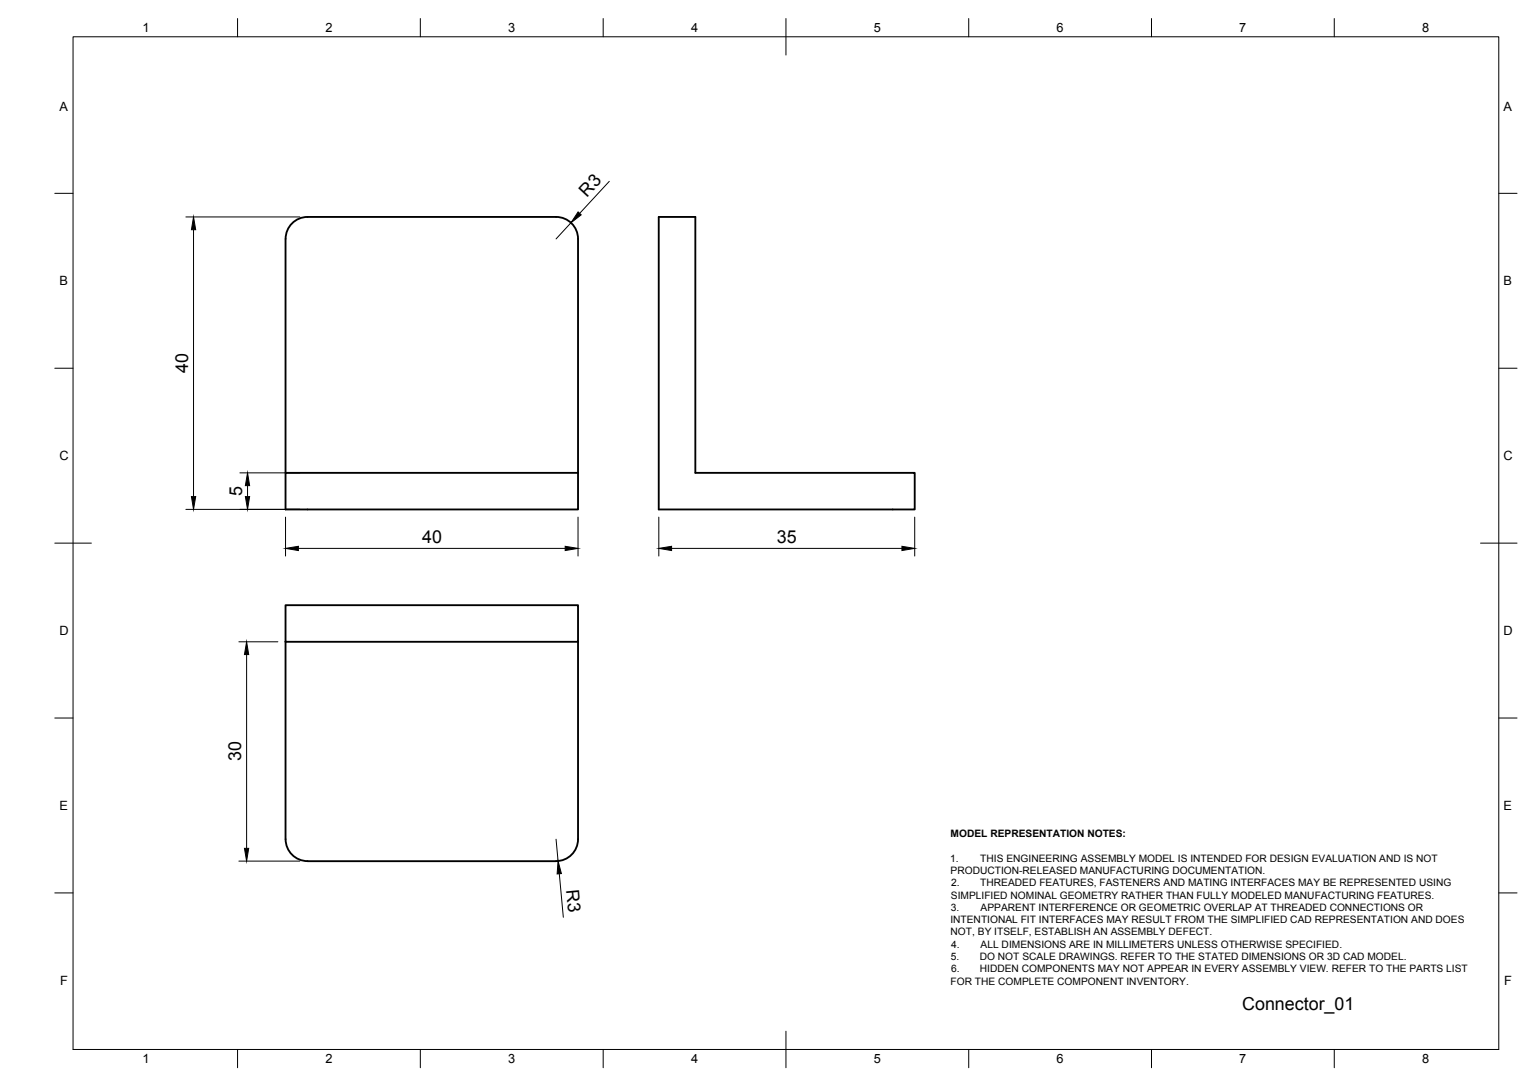
ISO-10303-21;
HEADER;
/* Generated by software containing ST-Developer
 * from STEP Tools, Inc. (www.steptools.com) 
 */

FILE_DESCRIPTION(
/* description */ (''),
/* implementation_level */ '2;1');

FILE_NAME(
/* name */ 'Connector_01.step',
/* time_stamp */ '2026-10-05T19:45:59-07:00',
/* author */ (''),
/* organization */ (''),
/* preprocessor_version */ 'ST-DEVELOPER v20.2',
/* originating_system */ 'Autodesk Translation Framework v15.15.0.0',
/* authorisation */ '');

FILE_SCHEMA (('AUTOMOTIVE_DESIGN { 1 0 10303 214 3 1 1 }'));
ENDSEC;

DATA;
#10=MECHANICAL_DESIGN_GEOMETRIC_PRESENTATION_REPRESENTATION('',(#91),#2462);
#73=SHAPE_REPRESENTATION_RELATIONSHIP('SRR','None',#2499,#82);
#82=ADVANCED_BREP_SHAPE_REPRESENTATION('',(#100),#2454);
#91=STYLED_ITEM('',(#2552),#100);
#100=MANIFOLD_SOLID_BREP('Body1',#1328);
#110=PLANE('',#1447);
#111=PLANE('',#1449);
#112=PLANE('',#1455);
#113=PLANE('',#1456);
#114=PLANE('',#1460);
#115=PLANE('',#1461);
#116=PLANE('',#1462);
#117=PLANE('',#1463);
#168=FACE_OUTER_BOUND('',#248,.T.);
#169=FACE_OUTER_BOUND('',#249,.T.);
#170=FACE_OUTER_BOUND('',#250,.T.);
#171=FACE_OUTER_BOUND('',#251,.T.);
#172=FACE_OUTER_BOUND('',#252,.T.);
#173=FACE_OUTER_BOUND('',#253,.T.);
#174=FACE_OUTER_BOUND('',#254,.T.);
#175=FACE_OUTER_BOUND('',#255,.T.);
#176=FACE_OUTER_BOUND('',#256,.T.);
#177=FACE_OUTER_BOUND('',#257,.T.);
#178=FACE_OUTER_BOUND('',#258,.T.);
#179=FACE_OUTER_BOUND('',#259,.T.);
#248=EDGE_LOOP('',(#900,#901,#902,#903));
#249=EDGE_LOOP('',(#904,#905,#906,#907,#908,#909));
#250=EDGE_LOOP('',(#910,#911,#912,#913));
#251=EDGE_LOOP('',(#914,#915,#916,#917));
#252=EDGE_LOOP('',(#918,#919,#920,#921));
#253=EDGE_LOOP('',(#922,#923,#924,#925));
#254=EDGE_LOOP('',(#926,#927,#928,#929,#930,#931));
#255=EDGE_LOOP('',(#932,#933,#934,#935));
#256=EDGE_LOOP('',(#936,#937,#938,#939,#940,#941));
#257=EDGE_LOOP('',(#942,#943,#944,#945,#946,#947));
#258=EDGE_LOOP('',(#948,#949,#950,#951,#952,#953));
#259=EDGE_LOOP('',(#954,#955,#956,#957,#958,#959));
#341=LINE('',#2000,#460);
#342=LINE('',#2003,#461);
#343=LINE('',#2006,#462);
#344=LINE('',#2010,#463);
#345=LINE('',#2012,#464);
#346=LINE('',#2013,#465);
#347=LINE('',#2016,#466);
#348=LINE('',#2017,#467);
#349=LINE('',#2021,#468);
#350=LINE('',#2027,#469);
#351=LINE('',#2030,#470);
#352=LINE('',#2033,#471);
#353=LINE('',#2035,#472);
#354=LINE('',#2036,#473);
#355=LINE('',#2039,#474);
#356=LINE('',#2041,#475);
#357=LINE('',#2043,#476);
#358=LINE('',#2048,#477);
#359=LINE('',#2050,#478);
#360=LINE('',#2051,#479);
#361=LINE('',#2053,#480);
#362=LINE('',#2055,#481);
#460=VECTOR('',#1600,10.);
#461=VECTOR('',#1603,10.);
#462=VECTOR('',#1606,10.);
#463=VECTOR('',#1609,10.);
#464=VECTOR('',#1610,10.);
#465=VECTOR('',#1611,10.);
#466=VECTOR('',#1614,10.);
#467=VECTOR('',#1615,10.);
#468=VECTOR('',#1620,10.);
#469=VECTOR('',#1625,10.);
#470=VECTOR('',#1628,10.);
#471=VECTOR('',#1631,10.);
#472=VECTOR('',#1632,10.);
#473=VECTOR('',#1633,10.);
#474=VECTOR('',#1636,10.);
#475=VECTOR('',#1637,10.);
#476=VECTOR('',#1638,10.);
#477=VECTOR('',#1645,10.);
#478=VECTOR('',#1648,10.);
#479=VECTOR('',#1649,10.);
#480=VECTOR('',#1652,10.);
#481=VECTOR('',#1655,10.);
#580=CIRCLE('',#1445,3.);
#581=CIRCLE('',#1446,3.);
#582=CIRCLE('',#1448,3.);
#583=CIRCLE('',#1451,3.);
#584=CIRCLE('',#1453,3.);
#585=CIRCLE('',#1454,3.);
#586=CIRCLE('',#1457,3.);
#587=CIRCLE('',#1459,3.);
#623=VERTEX_POINT('',#1996);
#624=VERTEX_POINT('',#1997);
#625=VERTEX_POINT('',#1999);
#626=VERTEX_POINT('',#2001);
#627=VERTEX_POINT('',#2005);
#628=VERTEX_POINT('',#2007);
#629=VERTEX_POINT('',#2009);
#630=VERTEX_POINT('',#2011);
#631=VERTEX_POINT('',#2015);
#632=VERTEX_POINT('',#2019);
#633=VERTEX_POINT('',#2023);
#634=VERTEX_POINT('',#2024);
#635=VERTEX_POINT('',#2026);
#636=VERTEX_POINT('',#2028);
#637=VERTEX_POINT('',#2032);
#638=VERTEX_POINT('',#2034);
#639=VERTEX_POINT('',#2038);
#640=VERTEX_POINT('',#2040);
#641=VERTEX_POINT('',#2042);
#642=VERTEX_POINT('',#2046);
#731=EDGE_CURVE('',#623,#624,#580,.T.);
#732=EDGE_CURVE('',#624,#625,#341,.T.);
#733=EDGE_CURVE('',#625,#626,#581,.T.);
#734=EDGE_CURVE('',#626,#623,#342,.T.);
#735=EDGE_CURVE('',#627,#625,#343,.T.);
#736=EDGE_CURVE('',#628,#627,#582,.T.);
#737=EDGE_CURVE('',#629,#628,#344,.T.);
#738=EDGE_CURVE('',#629,#630,#345,.T.);
#739=EDGE_CURVE('',#630,#626,#346,.T.);
#740=EDGE_CURVE('',#624,#631,#347,.T.);
#741=EDGE_CURVE('',#627,#631,#348,.T.);
#742=EDGE_CURVE('',#631,#632,#583,.T.);
#743=EDGE_CURVE('',#632,#628,#349,.T.);
#744=EDGE_CURVE('',#633,#634,#584,.T.);
#745=EDGE_CURVE('',#634,#635,#350,.T.);
#746=EDGE_CURVE('',#635,#636,#585,.T.);
#747=EDGE_CURVE('',#636,#633,#351,.T.);
#748=EDGE_CURVE('',#637,#636,#352,.T.);
#749=EDGE_CURVE('',#638,#637,#353,.T.);
#750=EDGE_CURVE('',#633,#638,#354,.T.);
#751=EDGE_CURVE('',#639,#635,#355,.T.);
#752=EDGE_CURVE('',#640,#639,#356,.T.);
#753=EDGE_CURVE('',#641,#640,#357,.T.);
#754=EDGE_CURVE('',#637,#641,#586,.T.);
#755=EDGE_CURVE('',#642,#638,#587,.T.);
#756=EDGE_CURVE('',#641,#642,#358,.T.);
#757=EDGE_CURVE('',#642,#630,#359,.T.);
#758=EDGE_CURVE('',#629,#634,#360,.T.);
#759=EDGE_CURVE('',#639,#632,#361,.T.);
#760=EDGE_CURVE('',#640,#623,#362,.T.);
#900=ORIENTED_EDGE('',*,*,#731,.T.);
#901=ORIENTED_EDGE('',*,*,#732,.T.);
#902=ORIENTED_EDGE('',*,*,#733,.T.);
#903=ORIENTED_EDGE('',*,*,#734,.T.);
#904=ORIENTED_EDGE('',*,*,#733,.F.);
#905=ORIENTED_EDGE('',*,*,#735,.F.);
#906=ORIENTED_EDGE('',*,*,#736,.F.);
#907=ORIENTED_EDGE('',*,*,#737,.F.);
#908=ORIENTED_EDGE('',*,*,#738,.T.);
#909=ORIENTED_EDGE('',*,*,#739,.T.);
#910=ORIENTED_EDGE('',*,*,#732,.F.);
#911=ORIENTED_EDGE('',*,*,#740,.T.);
#912=ORIENTED_EDGE('',*,*,#741,.F.);
#913=ORIENTED_EDGE('',*,*,#735,.T.);
#914=ORIENTED_EDGE('',*,*,#736,.T.);
#915=ORIENTED_EDGE('',*,*,#741,.T.);
#916=ORIENTED_EDGE('',*,*,#742,.T.);
#917=ORIENTED_EDGE('',*,*,#743,.T.);
#918=ORIENTED_EDGE('',*,*,#744,.T.);
#919=ORIENTED_EDGE('',*,*,#745,.T.);
#920=ORIENTED_EDGE('',*,*,#746,.T.);
#921=ORIENTED_EDGE('',*,*,#747,.T.);
#922=ORIENTED_EDGE('',*,*,#747,.F.);
#923=ORIENTED_EDGE('',*,*,#748,.F.);
#924=ORIENTED_EDGE('',*,*,#749,.F.);
#925=ORIENTED_EDGE('',*,*,#750,.F.);
#926=ORIENTED_EDGE('',*,*,#746,.F.);
#927=ORIENTED_EDGE('',*,*,#751,.F.);
#928=ORIENTED_EDGE('',*,*,#752,.F.);
#929=ORIENTED_EDGE('',*,*,#753,.F.);
#930=ORIENTED_EDGE('',*,*,#754,.F.);
#931=ORIENTED_EDGE('',*,*,#748,.T.);
#932=ORIENTED_EDGE('',*,*,#755,.T.);
#933=ORIENTED_EDGE('',*,*,#749,.T.);
#934=ORIENTED_EDGE('',*,*,#754,.T.);
#935=ORIENTED_EDGE('',*,*,#756,.T.);
#936=ORIENTED_EDGE('',*,*,#744,.F.);
#937=ORIENTED_EDGE('',*,*,#750,.T.);
#938=ORIENTED_EDGE('',*,*,#755,.F.);
#939=ORIENTED_EDGE('',*,*,#757,.T.);
#940=ORIENTED_EDGE('',*,*,#738,.F.);
#941=ORIENTED_EDGE('',*,*,#758,.T.);
#942=ORIENTED_EDGE('',*,*,#743,.F.);
#943=ORIENTED_EDGE('',*,*,#759,.F.);
#944=ORIENTED_EDGE('',*,*,#751,.T.);
#945=ORIENTED_EDGE('',*,*,#745,.F.);
#946=ORIENTED_EDGE('',*,*,#758,.F.);
#947=ORIENTED_EDGE('',*,*,#737,.T.);
#948=ORIENTED_EDGE('',*,*,#731,.F.);
#949=ORIENTED_EDGE('',*,*,#760,.F.);
#950=ORIENTED_EDGE('',*,*,#752,.T.);
#951=ORIENTED_EDGE('',*,*,#759,.T.);
#952=ORIENTED_EDGE('',*,*,#742,.F.);
#953=ORIENTED_EDGE('',*,*,#740,.F.);
#954=ORIENTED_EDGE('',*,*,#734,.F.);
#955=ORIENTED_EDGE('',*,*,#739,.F.);
#956=ORIENTED_EDGE('',*,*,#757,.F.);
#957=ORIENTED_EDGE('',*,*,#756,.F.);
#958=ORIENTED_EDGE('',*,*,#753,.T.);
#959=ORIENTED_EDGE('',*,*,#760,.T.);
#1227=CYLINDRICAL_SURFACE('',#1444,3.);
#1228=CYLINDRICAL_SURFACE('',#1450,3.);
#1229=CYLINDRICAL_SURFACE('',#1452,3.);
#1230=CYLINDRICAL_SURFACE('',#1458,3.);
#1250=ADVANCED_FACE('',(#168),#1227,.T.);
#1251=ADVANCED_FACE('',(#169),#110,.T.);
#1252=ADVANCED_FACE('',(#170),#111,.T.);
#1253=ADVANCED_FACE('',(#171),#1228,.T.);
#1254=ADVANCED_FACE('',(#172),#1229,.T.);
#1255=ADVANCED_FACE('',(#173),#112,.T.);
#1256=ADVANCED_FACE('',(#174),#113,.F.);
#1257=ADVANCED_FACE('',(#175),#1230,.T.);
#1258=ADVANCED_FACE('',(#176),#114,.T.);
#1259=ADVANCED_FACE('',(#177),#115,.T.);
#1260=ADVANCED_FACE('',(#178),#116,.T.);
#1261=ADVANCED_FACE('',(#179),#117,.T.);
#1328=CLOSED_SHELL('',(#1250,#1251,#1252,#1253,#1254,#1255,#1256,#1257,
#1258,#1259,#1260,#1261));
#1443=AXIS2_PLACEMENT_3D('',#1994,#1594,#1595);
#1444=AXIS2_PLACEMENT_3D('',#1995,#1596,#1597);
#1445=AXIS2_PLACEMENT_3D('',#1998,#1598,#1599);
#1446=AXIS2_PLACEMENT_3D('',#2002,#1601,#1602);
#1447=AXIS2_PLACEMENT_3D('',#2004,#1604,#1605);
#1448=AXIS2_PLACEMENT_3D('',#2008,#1607,#1608);
#1449=AXIS2_PLACEMENT_3D('',#2014,#1612,#1613);
#1450=AXIS2_PLACEMENT_3D('',#2018,#1616,#1617);
#1451=AXIS2_PLACEMENT_3D('',#2020,#1618,#1619);
#1452=AXIS2_PLACEMENT_3D('',#2022,#1621,#1622);
#1453=AXIS2_PLACEMENT_3D('',#2025,#1623,#1624);
#1454=AXIS2_PLACEMENT_3D('',#2029,#1626,#1627);
#1455=AXIS2_PLACEMENT_3D('',#2031,#1629,#1630);
#1456=AXIS2_PLACEMENT_3D('',#2037,#1634,#1635);
#1457=AXIS2_PLACEMENT_3D('',#2044,#1639,#1640);
#1458=AXIS2_PLACEMENT_3D('',#2045,#1641,#1642);
#1459=AXIS2_PLACEMENT_3D('',#2047,#1643,#1644);
#1460=AXIS2_PLACEMENT_3D('',#2049,#1646,#1647);
#1461=AXIS2_PLACEMENT_3D('',#2052,#1650,#1651);
#1462=AXIS2_PLACEMENT_3D('',#2054,#1653,#1654);
#1463=AXIS2_PLACEMENT_3D('',#2056,#1656,#1657);
#1594=DIRECTION('axis',(0.,0.,1.));
#1595=DIRECTION('refdir',(1.,0.,0.));
#1596=DIRECTION('center_axis',(0.,0.,-1.));
#1597=DIRECTION('ref_axis',(0.707106781186544,-0.707106781186551,0.));
#1598=DIRECTION('center_axis',(0.,0.,1.));
#1599=DIRECTION('ref_axis',(0.707106781186544,-0.707106781186551,0.));
#1600=DIRECTION('',(0.,0.,1.));
#1601=DIRECTION('center_axis',(0.,0.,-1.));
#1602=DIRECTION('ref_axis',(0.707106781186544,-0.707106781186551,0.));
#1603=DIRECTION('',(0.,0.,-1.));
#1604=DIRECTION('center_axis',(0.,0.,1.));
#1605=DIRECTION('ref_axis',(0.,-1.,0.));
#1606=DIRECTION('',(0.,-1.,0.));
#1607=DIRECTION('center_axis',(0.,0.,-1.));
#1608=DIRECTION('ref_axis',(0.707106781186544,0.707106781186551,0.));
#1609=DIRECTION('',(1.,0.,0.));
#1610=DIRECTION('',(0.,-1.,0.));
#1611=DIRECTION('',(1.,0.,0.));
#1612=DIRECTION('center_axis',(1.,0.,0.));
#1613=DIRECTION('ref_axis',(0.,0.,-1.));
#1614=DIRECTION('',(0.,1.,0.));
#1615=DIRECTION('',(0.,0.,-1.));
#1616=DIRECTION('center_axis',(0.,0.,1.));
#1617=DIRECTION('ref_axis',(0.707106781186544,0.707106781186551,0.));
#1618=DIRECTION('center_axis',(0.,0.,1.));
#1619=DIRECTION('ref_axis',(0.707106781186544,0.707106781186551,0.));
#1620=DIRECTION('',(0.,0.,1.));
#1621=DIRECTION('center_axis',(1.,0.,0.));
#1622=DIRECTION('ref_axis',(0.,0.707106781186547,0.707106781186547));
#1623=DIRECTION('center_axis',(-1.,0.,0.));
#1624=DIRECTION('ref_axis',(0.,0.707106781186547,0.707106781186547));
#1625=DIRECTION('',(-1.,0.,0.));
#1626=DIRECTION('center_axis',(1.,0.,0.));
#1627=DIRECTION('ref_axis',(0.,0.707106781186547,0.707106781186547));
#1628=DIRECTION('',(1.,0.,0.));
#1629=DIRECTION('center_axis',(0.,0.,1.));
#1630=DIRECTION('ref_axis',(0.,-1.,0.));
#1631=DIRECTION('',(0.,1.,0.));
#1632=DIRECTION('',(-1.,0.,0.));
#1633=DIRECTION('',(0.,-1.,0.));
#1634=DIRECTION('center_axis',(1.,0.,0.));
#1635=DIRECTION('ref_axis',(0.,1.,0.));
#1636=DIRECTION('',(0.,0.,1.));
#1637=DIRECTION('',(0.,1.,0.));
#1638=DIRECTION('',(0.,0.,-1.));
#1639=DIRECTION('center_axis',(1.,0.,0.));
#1640=DIRECTION('ref_axis',(0.,-0.707106781186547,0.707106781186547));
#1641=DIRECTION('center_axis',(1.,0.,0.));
#1642=DIRECTION('ref_axis',(0.,-0.707106781186547,0.707106781186547));
#1643=DIRECTION('center_axis',(-1.,0.,0.));
#1644=DIRECTION('ref_axis',(0.,-0.707106781186547,0.707106781186547));
#1645=DIRECTION('',(1.,0.,0.));
#1646=DIRECTION('center_axis',(1.,0.,0.));
#1647=DIRECTION('ref_axis',(0.,0.,-1.));
#1648=DIRECTION('',(0.,0.,-1.));
#1649=DIRECTION('',(0.,0.,1.));
#1650=DIRECTION('center_axis',(0.,1.,0.));
#1651=DIRECTION('ref_axis',(0.,0.,1.));
#1652=DIRECTION('',(1.,0.,0.));
#1653=DIRECTION('center_axis',(0.,0.,-1.));
#1654=DIRECTION('ref_axis',(0.,1.,0.));
#1655=DIRECTION('',(1.,0.,0.));
#1656=DIRECTION('center_axis',(0.,-1.,0.));
#1657=DIRECTION('ref_axis',(0.,0.,-1.));
#1994=CARTESIAN_POINT('',(0.,0.,0.));
#1995=CARTESIAN_POINT('Origin',(336.8,-17.,-16.25));
#1996=CARTESIAN_POINT('',(336.8,-20.,-20.));
#1997=CARTESIAN_POINT('',(339.8,-17.,-20.));
#1998=CARTESIAN_POINT('Origin',(336.8,-17.,-20.));
#1999=CARTESIAN_POINT('',(339.8,-17.,-15.));
#2000=CARTESIAN_POINT('',(339.8,-17.,-16.25));
#2001=CARTESIAN_POINT('',(336.8,-20.,-15.));
#2002=CARTESIAN_POINT('Origin',(336.8,-17.,-15.));
#2003=CARTESIAN_POINT('',(336.8,-20.,-16.25));
#2004=CARTESIAN_POINT('Origin',(304.8,20.,-15.));
#2005=CARTESIAN_POINT('',(339.8,17.,-15.));
#2006=CARTESIAN_POINT('',(339.8,20.,-15.));
#2007=CARTESIAN_POINT('',(336.8,20.,-15.));
#2008=CARTESIAN_POINT('Origin',(336.8,17.,-15.));
#2009=CARTESIAN_POINT('',(309.8,20.,-15.));
#2010=CARTESIAN_POINT('',(304.8,20.,-15.));
#2011=CARTESIAN_POINT('',(309.8,-20.,-15.));
#2012=CARTESIAN_POINT('',(309.8,10.,-15.));
#2013=CARTESIAN_POINT('',(304.8,-20.,-15.));
#2014=CARTESIAN_POINT('Origin',(339.8,0.,-17.5));
#2015=CARTESIAN_POINT('',(339.8,17.,-20.));
#2016=CARTESIAN_POINT('',(339.8,-20.,-20.));
#2017=CARTESIAN_POINT('',(339.8,17.,-18.75));
#2018=CARTESIAN_POINT('Origin',(336.8,17.,-18.75));
#2019=CARTESIAN_POINT('',(336.8,20.,-20.));
#2020=CARTESIAN_POINT('Origin',(336.8,17.,-20.));
#2021=CARTESIAN_POINT('',(336.8,20.,-18.75));
#2022=CARTESIAN_POINT('Origin',(304.8,17.,17.));
#2023=CARTESIAN_POINT('',(309.8,17.,20.));
#2024=CARTESIAN_POINT('',(309.8,20.,17.));
#2025=CARTESIAN_POINT('Origin',(309.8,17.,17.));
#2026=CARTESIAN_POINT('',(304.8,20.,17.));
#2027=CARTESIAN_POINT('',(304.8,20.,17.));
#2028=CARTESIAN_POINT('',(304.8,17.,20.));
#2029=CARTESIAN_POINT('Origin',(304.8,17.,17.));
#2030=CARTESIAN_POINT('',(304.8,17.,20.));
#2031=CARTESIAN_POINT('Origin',(304.8,20.,20.));
#2032=CARTESIAN_POINT('',(304.8,-17.,20.));
#2033=CARTESIAN_POINT('',(304.8,-20.,20.));
#2034=CARTESIAN_POINT('',(309.8,-17.,20.));
#2035=CARTESIAN_POINT('',(304.8,-17.,20.));
#2036=CARTESIAN_POINT('',(309.8,-20.,20.));
#2037=CARTESIAN_POINT('Origin',(304.8,0.,-17.5));
#2038=CARTESIAN_POINT('',(304.8,20.,-20.));
#2039=CARTESIAN_POINT('',(304.8,20.,-20.));
#2040=CARTESIAN_POINT('',(304.8,-20.,-20.));
#2041=CARTESIAN_POINT('',(304.8,-20.,-20.));
#2042=CARTESIAN_POINT('',(304.8,-20.,17.));
#2043=CARTESIAN_POINT('',(304.8,-20.,-15.));
#2044=CARTESIAN_POINT('Origin',(304.8,-17.,17.));
#2045=CARTESIAN_POINT('Origin',(304.8,-17.,17.));
#2046=CARTESIAN_POINT('',(309.8,-20.,17.));
#2047=CARTESIAN_POINT('Origin',(309.8,-17.,17.));
#2048=CARTESIAN_POINT('',(304.8,-20.,17.));
#2049=CARTESIAN_POINT('Origin',(309.8,0.,2.5));
#2050=CARTESIAN_POINT('',(309.8,-20.,-20.));
#2051=CARTESIAN_POINT('',(309.8,20.,20.));
#2052=CARTESIAN_POINT('Origin',(304.8,20.,-20.));
#2053=CARTESIAN_POINT('',(304.8,20.,-20.));
#2054=CARTESIAN_POINT('Origin',(304.8,-20.,-20.));
#2055=CARTESIAN_POINT('',(304.8,-20.,-20.));
#2056=CARTESIAN_POINT('Origin',(304.8,-20.,-15.));
#2443=UNCERTAINTY_MEASURE_WITH_UNIT(LENGTH_MEASURE(0.01),#2463,
'DISTANCE_ACCURACY_VALUE',
'Maximum model space distance between geometric entities at asserted c
onnectivities');
#2451=UNCERTAINTY_MEASURE_WITH_UNIT(LENGTH_MEASURE(0.01),#2463,
'DISTANCE_ACCURACY_VALUE',
'Maximum model space distance between geometric entities at asserted c
onnectivities');
#2454=(
GEOMETRIC_REPRESENTATION_CONTEXT(3)
GLOBAL_UNCERTAINTY_ASSIGNED_CONTEXT((#2443))
GLOBAL_UNIT_ASSIGNED_CONTEXT((#2463,#2465,#2466))
REPRESENTATION_CONTEXT('','3D')
);
#2462=(
GEOMETRIC_REPRESENTATION_CONTEXT(3)
GLOBAL_UNCERTAINTY_ASSIGNED_CONTEXT((#2451))
GLOBAL_UNIT_ASSIGNED_CONTEXT((#2463,#2465,#2466))
REPRESENTATION_CONTEXT('','3D')
);
#2463=(
LENGTH_UNIT()
NAMED_UNIT(*)
SI_UNIT(.MILLI.,.METRE.)
);
#2465=(
NAMED_UNIT(*)
PLANE_ANGLE_UNIT()
SI_UNIT($,.RADIAN.)
);
#2466=(
NAMED_UNIT(*)
SI_UNIT($,.STERADIAN.)
SOLID_ANGLE_UNIT()
);
#2469=SHAPE_DEFINITION_REPRESENTATION(#2479,#2499);
#2479=PRODUCT_DEFINITION_SHAPE('',$,#2510);
#2499=SHAPE_REPRESENTATION('',(#1443),#2454);
#2507=PRODUCT_DEFINITION_CONTEXT('part definition',#2539,'design');
#2510=PRODUCT_DEFINITION('Connector_01','Connector_01',#2520,#2507);
#2520=PRODUCT_DEFINITION_FORMATION('',$,#2543);
#2539=APPLICATION_CONTEXT(
'Core Data for Automotive Mechanical Design Process');
#2540=PRODUCT_CONTEXT('part definition',#2539,'mechanical');
#2543=PRODUCT('Connector_01','Connector_01',$,(#2540));
#2552=PRESENTATION_STYLE_ASSIGNMENT((#2555));
#2555=SURFACE_STYLE_USAGE(.BOTH.,#2558);
#2558=SURFACE_SIDE_STYLE('',(#2561));
#2561=SURFACE_STYLE_FILL_AREA(#2564);
#2564=FILL_AREA_STYLE('Opaque(160,160,160)',(#2567));
#2567=FILL_AREA_STYLE_COLOUR('Opaque(160,160,160)',#2570);
#2570=COLOUR_RGB('Opaque(160,160,160)', 0.09019608, 0.27058824, 0.51372549);
ENDSEC;
END-ISO-10303-21;
